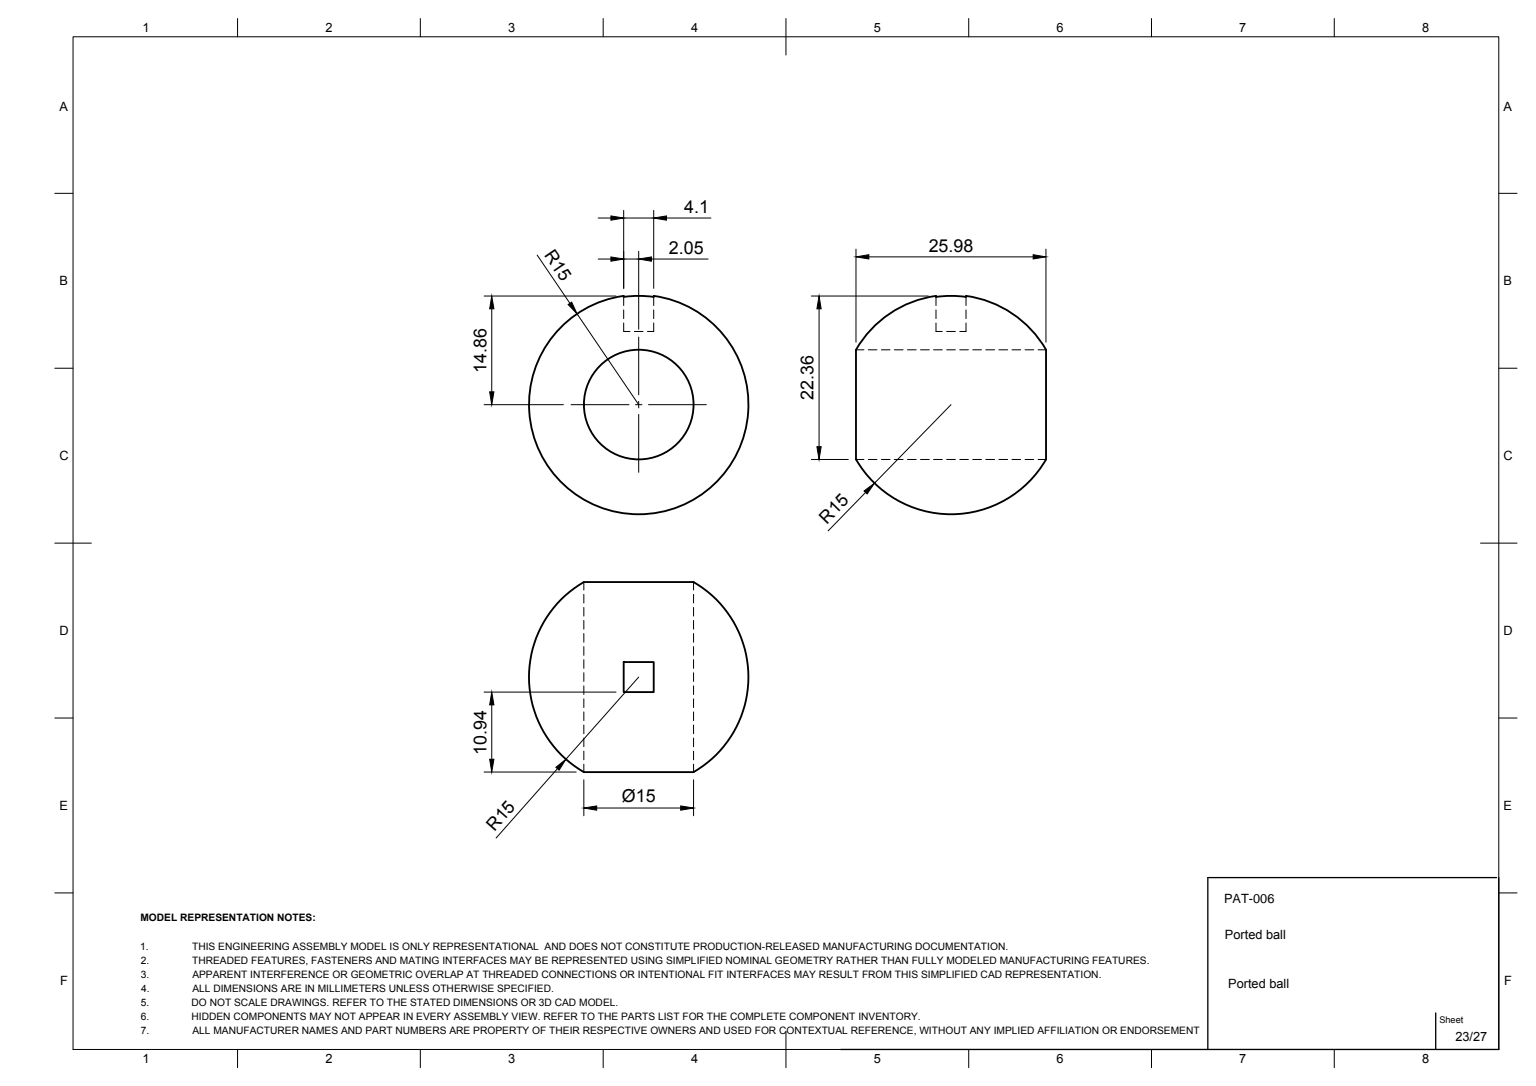
ISO-10303-21;
HEADER;
/* Generated by software containing ST-Developer
 * from STEP Tools, Inc. (www.steptools.com) 
 */

FILE_DESCRIPTION(
/* description */ ('Ball-type isolation valve (generic)'),
/* implementation_level */ '2;1');

FILE_NAME(
/* name */ 'Ported ball.step',
/* time_stamp */ '2026-10-27T10:53:05-07:00',
/* author */ (''),
/* organization */ (''),
/* preprocessor_version */ 'ST-DEVELOPER v20.2',
/* originating_system */ 'Autodesk Translation Framework v15.17.0.0',
/* authorisation */ '');

FILE_SCHEMA (('AUTOMOTIVE_DESIGN { 1 0 10303 214 3 1 1 }'));
ENDSEC;

DATA;
#10=MECHANICAL_DESIGN_GEOMETRIC_PRESENTATION_REPRESENTATION('',(#297),#7425);
#245=SHAPE_REPRESENTATION_RELATIONSHIP('SRR','None',#7556,#271);
#271=ADVANCED_BREP_SHAPE_REPRESENTATION('',(#321),#7419);
#297=STYLED_ITEM('',(#7730),#321);
#321=MANIFOLD_SOLID_BREP('Body1',#4104);
#330=SPHERICAL_SURFACE('',#4800,1.5);
#410=FACE_BOUND('',#1098,.T.);
#411=FACE_BOUND('',#1099,.T.);
#525=PLANE('',#4787);
#526=PLANE('',#4789);
#527=PLANE('',#4792);
#528=PLANE('',#4794);
#529=PLANE('',#4796);
#763=FACE_OUTER_BOUND('',#1091,.T.);
#764=FACE_OUTER_BOUND('',#1092,.T.);
#765=FACE_OUTER_BOUND('',#1093,.T.);
#766=FACE_OUTER_BOUND('',#1094,.T.);
#767=FACE_OUTER_BOUND('',#1095,.T.);
#768=FACE_OUTER_BOUND('',#1096,.T.);
#769=FACE_OUTER_BOUND('',#1097,.T.);
#1091=EDGE_LOOP('',(#3495,#3496,#3497,#3498));
#1092=EDGE_LOOP('',(#3499,#3500,#3501,#3502,#3503));
#1093=EDGE_LOOP('',(#3504,#3505,#3506,#3507));
#1094=EDGE_LOOP('',(#3508,#3509,#3510,#3511));
#1095=EDGE_LOOP('',(#3512,#3513,#3514,#3515));
#1096=EDGE_LOOP('',(#3516,#3517,#3518,#3519));
#1097=EDGE_LOOP('',(#3520,#3521,#3522,#3523,#3524,#3525,#3526));
#1098=EDGE_LOOP('',(#3527));
#1099=EDGE_LOOP('',(#3528));
#1369=LINE('',#7071,#1677);
#1370=LINE('',#7073,#1678);
#1371=LINE('',#7074,#1679);
#1372=LINE('',#7079,#1680);
#1373=LINE('',#7081,#1681);
#1374=LINE('',#7087,#1682);
#1375=LINE('',#7088,#1683);
#1376=LINE('',#7091,#1684);
#1377=LINE('',#7097,#1685);
#1677=VECTOR('',#5882,1.);
#1678=VECTOR('',#5883,1.);
#1679=VECTOR('',#5884,1.);
#1680=VECTOR('',#5889,1.);
#1681=VECTOR('',#5890,1.);
#1682=VECTOR('',#5897,1.);
#1683=VECTOR('',#5898,1.);
#1684=VECTOR('',#5903,1.);
#1685=VECTOR('',#5910,0.75);
#1925=CIRCLE('',#4788,1.48592563743951);
#1926=CIRCLE('',#4790,1.48592563743951);
#1927=CIRCLE('',#4791,1.48592563743951);
#1928=CIRCLE('',#4793,1.48592563743951);
#1929=CIRCLE('',#4795,1.48592563743951);
#1930=CIRCLE('',#4798,0.75);
#1931=CIRCLE('',#4799,0.75);
#1932=CIRCLE('',#4801,1.5);
#2193=VERTEX_POINT('',#7067);
#2194=VERTEX_POINT('',#7068);
#2195=VERTEX_POINT('',#7070);
#2196=VERTEX_POINT('',#7072);
#2197=VERTEX_POINT('',#7076);
#2198=VERTEX_POINT('',#7078);
#2199=VERTEX_POINT('',#7080);
#2200=VERTEX_POINT('',#7084);
#2201=VERTEX_POINT('',#7086);
#2202=VERTEX_POINT('',#7094);
#2203=VERTEX_POINT('',#7096);
#2204=VERTEX_POINT('',#7100);
#2640=EDGE_CURVE('',#2193,#2194,#1925,.T.);
#2641=EDGE_CURVE('',#2195,#2193,#1369,.T.);
#2642=EDGE_CURVE('',#2196,#2195,#1370,.T.);
#2643=EDGE_CURVE('',#2196,#2194,#1371,.T.);
#2644=EDGE_CURVE('',#2194,#2197,#1926,.T.);
#2645=EDGE_CURVE('',#2198,#2196,#1372,.T.);
#2646=EDGE_CURVE('',#2198,#2199,#1373,.T.);
#2647=EDGE_CURVE('',#2197,#2199,#1927,.T.);
#2648=EDGE_CURVE('',#2199,#2200,#1928,.T.);
#2649=EDGE_CURVE('',#2201,#2198,#1374,.T.);
#2650=EDGE_CURVE('',#2201,#2200,#1375,.T.);
#2651=EDGE_CURVE('',#2200,#2193,#1929,.T.);
#2652=EDGE_CURVE('',#2195,#2201,#1376,.T.);
#2653=EDGE_CURVE('',#2202,#2202,#1930,.T.);
#2654=EDGE_CURVE('',#2202,#2203,#1377,.T.);
#2655=EDGE_CURVE('',#2203,#2203,#1931,.T.);
#2656=EDGE_CURVE('',#2197,#2204,#1932,.T.);
#3495=ORIENTED_EDGE('',*,*,#2640,.F.);
#3496=ORIENTED_EDGE('',*,*,#2641,.F.);
#3497=ORIENTED_EDGE('',*,*,#2642,.F.);
#3498=ORIENTED_EDGE('',*,*,#2643,.T.);
#3499=ORIENTED_EDGE('',*,*,#2644,.F.);
#3500=ORIENTED_EDGE('',*,*,#2643,.F.);
#3501=ORIENTED_EDGE('',*,*,#2645,.F.);
#3502=ORIENTED_EDGE('',*,*,#2646,.T.);
#3503=ORIENTED_EDGE('',*,*,#2647,.F.);
#3504=ORIENTED_EDGE('',*,*,#2648,.F.);
#3505=ORIENTED_EDGE('',*,*,#2646,.F.);
#3506=ORIENTED_EDGE('',*,*,#2649,.F.);
#3507=ORIENTED_EDGE('',*,*,#2650,.T.);
#3508=ORIENTED_EDGE('',*,*,#2651,.F.);
#3509=ORIENTED_EDGE('',*,*,#2650,.F.);
#3510=ORIENTED_EDGE('',*,*,#2652,.F.);
#3511=ORIENTED_EDGE('',*,*,#2641,.T.);
#3512=ORIENTED_EDGE('',*,*,#2645,.T.);
#3513=ORIENTED_EDGE('',*,*,#2642,.T.);
#3514=ORIENTED_EDGE('',*,*,#2652,.T.);
#3515=ORIENTED_EDGE('',*,*,#2649,.T.);
#3516=ORIENTED_EDGE('',*,*,#2653,.F.);
#3517=ORIENTED_EDGE('',*,*,#2654,.T.);
#3518=ORIENTED_EDGE('',*,*,#2655,.F.);
#3519=ORIENTED_EDGE('',*,*,#2654,.F.);
#3520=ORIENTED_EDGE('',*,*,#2648,.T.);
#3521=ORIENTED_EDGE('',*,*,#2651,.T.);
#3522=ORIENTED_EDGE('',*,*,#2640,.T.);
#3523=ORIENTED_EDGE('',*,*,#2644,.T.);
#3524=ORIENTED_EDGE('',*,*,#2656,.T.);
#3525=ORIENTED_EDGE('',*,*,#2656,.F.);
#3526=ORIENTED_EDGE('',*,*,#2647,.T.);
#3527=ORIENTED_EDGE('',*,*,#2655,.T.);
#3528=ORIENTED_EDGE('',*,*,#2653,.T.);
#3826=CYLINDRICAL_SURFACE('',#4797,0.75);
#4017=ADVANCED_FACE('',(#763),#525,.F.);
#4018=ADVANCED_FACE('',(#764),#526,.F.);
#4019=ADVANCED_FACE('',(#765),#527,.F.);
#4020=ADVANCED_FACE('',(#766),#528,.F.);
#4021=ADVANCED_FACE('',(#767),#529,.T.);
#4022=ADVANCED_FACE('',(#768),#3826,.F.);
#4023=ADVANCED_FACE('',(#769,#410,#411),#330,.T.);
#4104=CLOSED_SHELL('',(#4017,#4018,#4019,#4020,#4021,#4022,#4023));
#4786=AXIS2_PLACEMENT_3D('',#7065,#5876,#5877);
#4787=AXIS2_PLACEMENT_3D('',#7066,#5878,#5879);
#4788=AXIS2_PLACEMENT_3D('',#7069,#5880,#5881);
#4789=AXIS2_PLACEMENT_3D('',#7075,#5885,#5886);
#4790=AXIS2_PLACEMENT_3D('',#7077,#5887,#5888);
#4791=AXIS2_PLACEMENT_3D('',#7082,#5891,#5892);
#4792=AXIS2_PLACEMENT_3D('',#7083,#5893,#5894);
#4793=AXIS2_PLACEMENT_3D('',#7085,#5895,#5896);
#4794=AXIS2_PLACEMENT_3D('',#7089,#5899,#5900);
#4795=AXIS2_PLACEMENT_3D('',#7090,#5901,#5902);
#4796=AXIS2_PLACEMENT_3D('',#7092,#5904,#5905);
#4797=AXIS2_PLACEMENT_3D('',#7093,#5906,#5907);
#4798=AXIS2_PLACEMENT_3D('',#7095,#5908,#5909);
#4799=AXIS2_PLACEMENT_3D('',#7098,#5911,#5912);
#4800=AXIS2_PLACEMENT_3D('',#7099,#5913,#5914);
#4801=AXIS2_PLACEMENT_3D('',#7101,#5915,#5916);
#5876=DIRECTION('axis',(0.,0.,1.));
#5877=DIRECTION('refdir',(1.,0.,0.));
#5878=DIRECTION('center_axis',(0.,-1.,0.));
#5879=DIRECTION('ref_axis',(1.,0.,0.));
#5880=DIRECTION('center_axis',(0.,-1.,0.));
#5881=DIRECTION('ref_axis',(0.,0.,1.));
#5882=DIRECTION('',(0.,0.,1.));
#5883=DIRECTION('',(1.,0.,0.));
#5884=DIRECTION('',(0.,0.,1.));
#5885=DIRECTION('center_axis',(-1.,0.,0.));
#5886=DIRECTION('ref_axis',(0.,-1.,0.));
#5887=DIRECTION('center_axis',(-1.,0.,0.));
#5888=DIRECTION('ref_axis',(0.,0.,-1.));
#5889=DIRECTION('',(0.,-1.,0.));
#5890=DIRECTION('',(0.,0.,1.));
#5891=DIRECTION('center_axis',(-1.,0.,0.));
#5892=DIRECTION('ref_axis',(0.,0.,-1.));
#5893=DIRECTION('center_axis',(0.,1.,0.));
#5894=DIRECTION('ref_axis',(-1.,0.,0.));
#5895=DIRECTION('center_axis',(0.,1.,0.));
#5896=DIRECTION('ref_axis',(0.,0.,-1.));
#5897=DIRECTION('',(-1.,0.,0.));
#5898=DIRECTION('',(0.,0.,1.));
#5899=DIRECTION('center_axis',(1.,0.,0.));
#5900=DIRECTION('ref_axis',(0.,1.,0.));
#5901=DIRECTION('center_axis',(1.,0.,0.));
#5902=DIRECTION('ref_axis',(0.,0.,1.));
#5903=DIRECTION('',(0.,1.,0.));
#5904=DIRECTION('center_axis',(0.,0.,1.));
#5905=DIRECTION('ref_axis',(1.,0.,0.));
#5906=DIRECTION('center_axis',(0.,1.,0.));
#5907=DIRECTION('ref_axis',(1.,0.,0.));
#5908=DIRECTION('center_axis',(0.,1.,0.));
#5909=DIRECTION('ref_axis',(1.,0.,0.));
#5910=DIRECTION('',(0.,1.,0.));
#5911=DIRECTION('center_axis',(0.,-1.,0.));
#5912=DIRECTION('ref_axis',(1.,0.,0.));
#5913=DIRECTION('center_axis',(6.12323399573677E-17,0.,1.));
#5914=DIRECTION('ref_axis',(1.,0.,0.));
#5915=DIRECTION('center_axis',(1.22464679914735E-16,-1.,0.));
#5916=DIRECTION('ref_axis',(-1.,-1.22464679914735E-16,0.));
#7065=CARTESIAN_POINT('',(0.,0.,0.));
#7066=CARTESIAN_POINT('Origin',(-0.205,-0.205,6.));
#7067=CARTESIAN_POINT('',(0.205,-0.205,6.47171668469172));
#7068=CARTESIAN_POINT('',(-0.205,-0.205,6.47171668469172));
#7069=CARTESIAN_POINT('Origin',(0.,-0.205,5.));
#7070=CARTESIAN_POINT('',(0.205,-0.205,6.));
#7071=CARTESIAN_POINT('',(0.205,-0.205,6.));
#7072=CARTESIAN_POINT('',(-0.205,-0.205,6.));
#7073=CARTESIAN_POINT('',(-0.205,-0.205,6.));
#7074=CARTESIAN_POINT('',(-0.205,-0.205,6.));
#7075=CARTESIAN_POINT('Origin',(-0.205,0.205,6.));
#7076=CARTESIAN_POINT('',(-0.205,-2.51052593825207E-17,6.48592563743951));
#7077=CARTESIAN_POINT('Origin',(-0.205,0.,5.));
#7078=CARTESIAN_POINT('',(-0.205,0.205,6.));
#7079=CARTESIAN_POINT('',(-0.205,0.205,6.));
#7080=CARTESIAN_POINT('',(-0.205,0.205,6.47171668469172));
#7081=CARTESIAN_POINT('',(-0.205,0.205,6.));
#7082=CARTESIAN_POINT('Origin',(-0.205,0.,5.));
#7083=CARTESIAN_POINT('Origin',(0.205,0.205,6.));
#7084=CARTESIAN_POINT('',(0.205,0.205,6.47171668469172));
#7085=CARTESIAN_POINT('Origin',(0.,0.205,5.));
#7086=CARTESIAN_POINT('',(0.205,0.205,6.));
#7087=CARTESIAN_POINT('',(0.205,0.205,6.));
#7088=CARTESIAN_POINT('',(0.205,0.205,6.));
#7089=CARTESIAN_POINT('Origin',(0.205,-0.205,6.));
#7090=CARTESIAN_POINT('Origin',(0.205,0.,5.));
#7091=CARTESIAN_POINT('',(0.205,-0.205,6.));
#7092=CARTESIAN_POINT('Origin',(0.,0.,6.));
#7093=CARTESIAN_POINT('Origin',(0.,-1.6,5.));
#7094=CARTESIAN_POINT('',(-0.75,-1.29903810567666,5.));
#7095=CARTESIAN_POINT('Origin',(0.,-1.29903810567666,5.));
#7096=CARTESIAN_POINT('',(-0.75,1.29903810567666,5.));
#7097=CARTESIAN_POINT('',(-0.75,-1.6,5.));
#7098=CARTESIAN_POINT('Origin',(0.,1.29903810567666,5.));
#7099=CARTESIAN_POINT('Origin',(0.,0.,5.));
#7100=CARTESIAN_POINT('',(-9.18485099360515E-17,-1.12481983699639E-32,3.5));
#7101=CARTESIAN_POINT('Origin',(0.,0.,5.));
#7389=UNCERTAINTY_MEASURE_WITH_UNIT(LENGTH_MEASURE(0.001),#7426,
'DISTANCE_ACCURACY_VALUE',
'Maximum model space distance between geometric entities at asserted c
onnectivities');
#7395=UNCERTAINTY_MEASURE_WITH_UNIT(LENGTH_MEASURE(0.001),#7426,
'DISTANCE_ACCURACY_VALUE',
'Maximum model space distance between geometric entities at asserted c
onnectivities');
#7419=(
GEOMETRIC_REPRESENTATION_CONTEXT(3)
GLOBAL_UNCERTAINTY_ASSIGNED_CONTEXT((#7389))
GLOBAL_UNIT_ASSIGNED_CONTEXT((#7426,#7428,#7429))
REPRESENTATION_CONTEXT('','3D')
);
#7425=(
GEOMETRIC_REPRESENTATION_CONTEXT(3)
GLOBAL_UNCERTAINTY_ASSIGNED_CONTEXT((#7395))
GLOBAL_UNIT_ASSIGNED_CONTEXT((#7426,#7428,#7429))
REPRESENTATION_CONTEXT('','3D')
);
#7426=(
LENGTH_UNIT()
NAMED_UNIT(*)
SI_UNIT(.CENTI.,.METRE.)
);
#7428=(
NAMED_UNIT(*)
PLANE_ANGLE_UNIT()
SI_UNIT($,.RADIAN.)
);
#7429=(
NAMED_UNIT(*)
SI_UNIT($,.STERADIAN.)
SOLID_ANGLE_UNIT()
);
#7453=SHAPE_DEFINITION_REPRESENTATION(#7519,#7556);
#7519=PRODUCT_DEFINITION_SHAPE('',$,#7586);
#7556=SHAPE_REPRESENTATION('',(#4786),#7419);
#7562=PRODUCT_DEFINITION_CONTEXT('part definition',#7651,'design');
#7586=PRODUCT_DEFINITION('Ported ball','Ported ball',#7615,#7562);
#7615=PRODUCT_DEFINITION_FORMATION('',$,#7676);
#7651=APPLICATION_CONTEXT(
'Core Data for Automotive Mechanical Design Process');
#7652=PRODUCT_CONTEXT('part definition',#7651,'mechanical');
#7676=PRODUCT('Ported ball','Ported ball','Ported ball',(#7652));
#7724=COLOUR_RGB('Light Blue',0.38,0.62,0.78);
#7725=FILL_AREA_STYLE_COLOUR('',#7724);
#7726=FILL_AREA_STYLE('',(#7725));
#7727=SURFACE_STYLE_FILL_AREA(#7726);
#7728=SURFACE_SIDE_STYLE('',(#7727));
#7729=SURFACE_STYLE_USAGE(.BOTH.,#7728);
#7730=PRESENTATION_STYLE_ASSIGNMENT((#7729));
ENDSEC;
END-ISO-10303-21;
